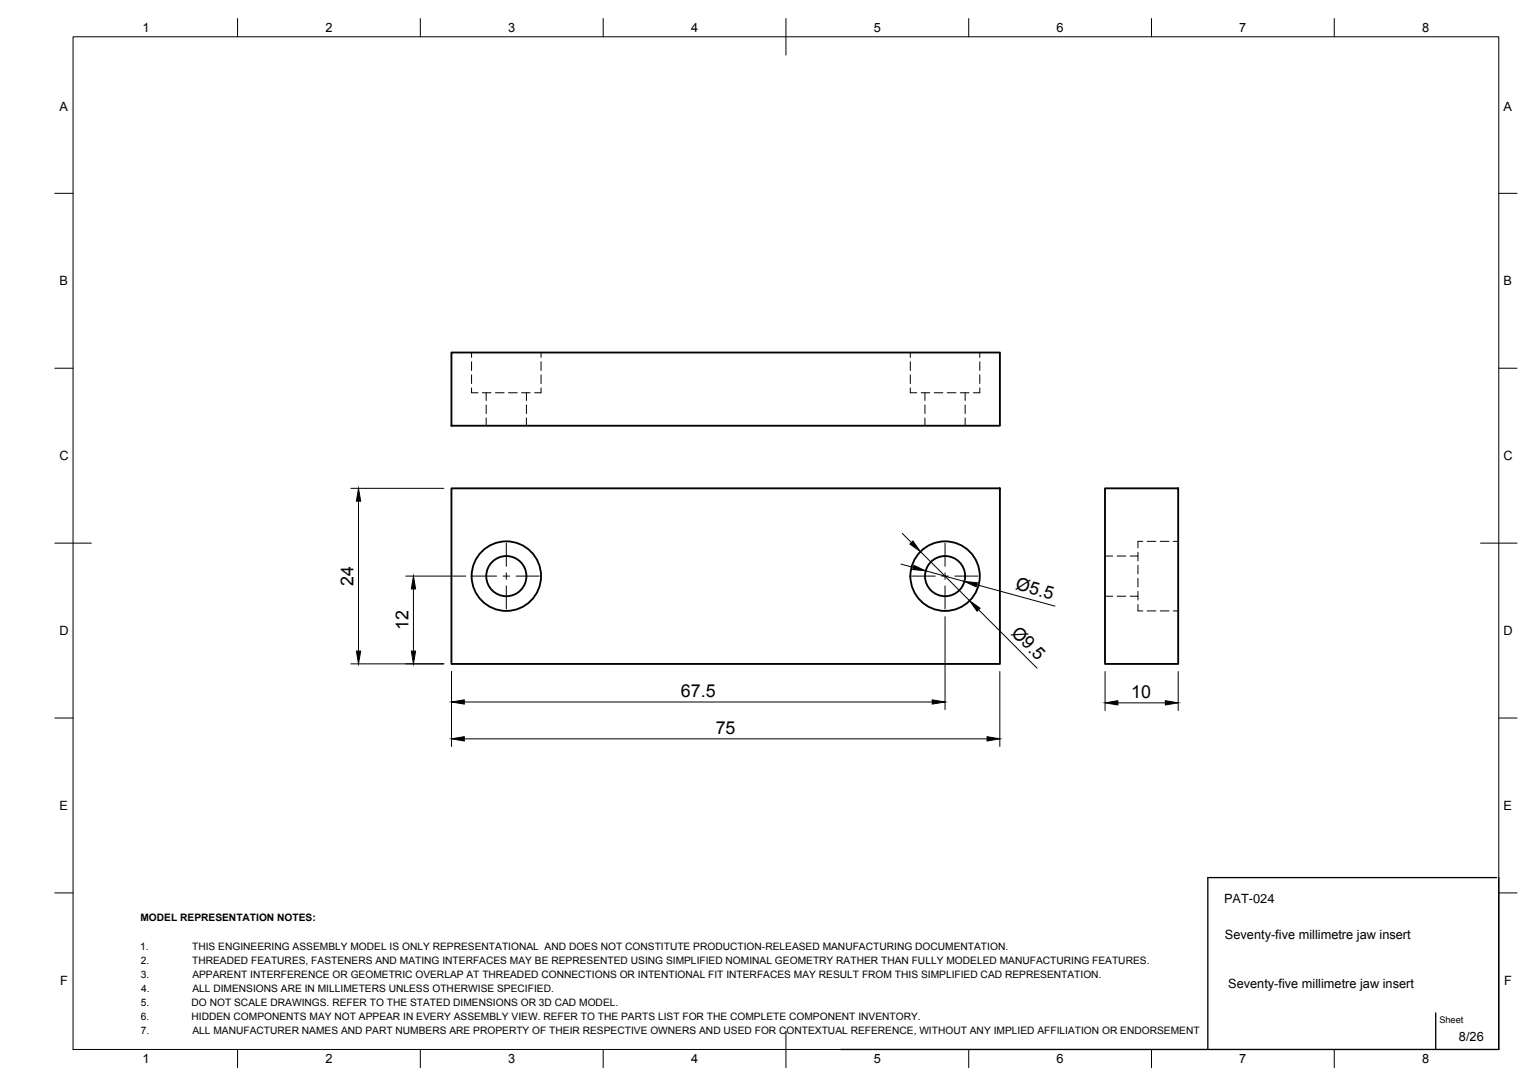
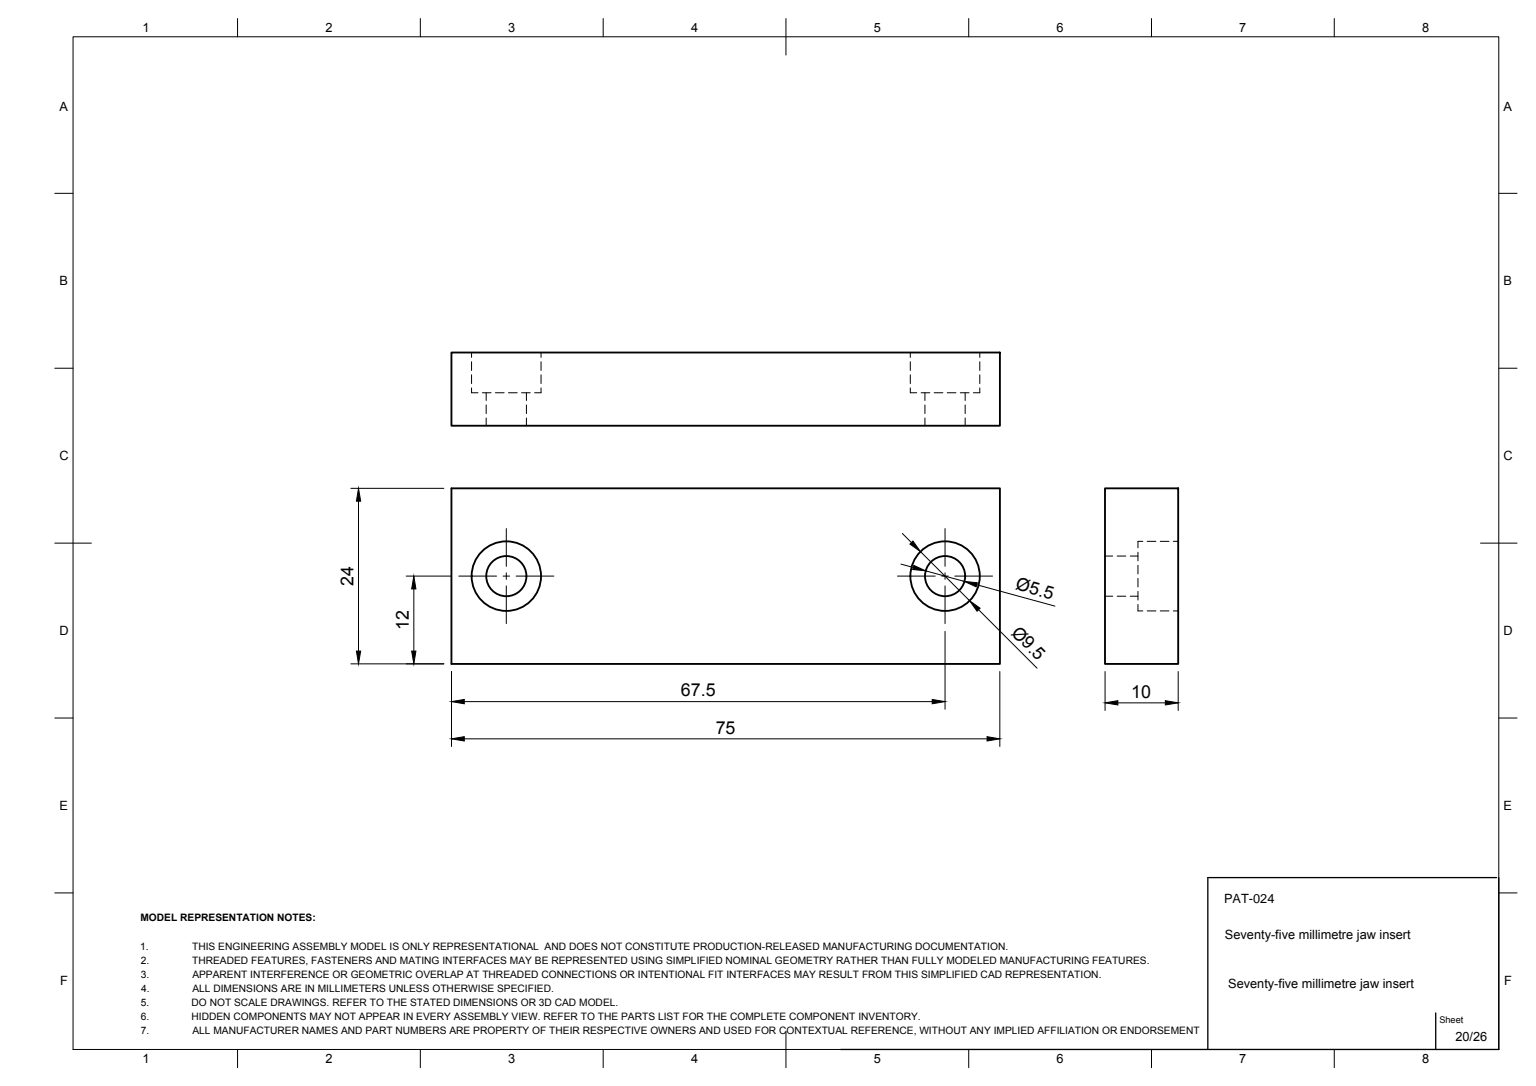
ISO-10303-21;
HEADER;
/* Generated by software containing ST-Developer
 * from STEP Tools, Inc. (www.steptools.com) 
 */

FILE_DESCRIPTION(
/* description */ ('Compact handwheel screw vise'),
/* implementation_level */ '2;1');

FILE_NAME(
/* name */ 'Seventy-five millimetre jaw insert.step',
/* time_stamp */ '2026-10-29T16:08:22-07:00',
/* author */ (''),
/* organization */ (''),
/* preprocessor_version */ 'ST-DEVELOPER v20.2',
/* originating_system */ 'Autodesk Translation Framework v15.17.0.0',
/* authorisation */ '');

FILE_SCHEMA (('AUTOMOTIVE_DESIGN { 1 0 10303 214 3 1 1 }'));
ENDSEC;

DATA;
#10=MECHANICAL_DESIGN_GEOMETRIC_PRESENTATION_REPRESENTATION('',(#649),#25074);
#593=SHAPE_REPRESENTATION_RELATIONSHIP('SRR','None',#25201,#621);
#621=ADVANCED_BREP_SHAPE_REPRESENTATION('',(#685),#25048);
#649=STYLED_ITEM('',(#25453),#685);
#685=MANIFOLD_SOLID_BREP('Body1',#8057);
#753=FACE_BOUND('',#1590,.T.);
#754=FACE_BOUND('',#1591,.T.);
#755=FACE_BOUND('',#1595,.T.);
#756=FACE_BOUND('',#1596,.T.);
#757=FACE_BOUND('',#1599,.T.);
#758=FACE_BOUND('',#1602,.T.);
#860=PLANE('',#8528);
#861=PLANE('',#8529);
#862=PLANE('',#8532);
#863=PLANE('',#8533);
#864=PLANE('',#8534);
#865=PLANE('',#8539);
#866=PLANE('',#8543);
#867=PLANE('',#8547);
#1077=FACE_OUTER_BOUND('',#1588,.T.);
#1078=FACE_OUTER_BOUND('',#1589,.T.);
#1079=FACE_OUTER_BOUND('',#1592,.T.);
#1080=FACE_OUTER_BOUND('',#1593,.T.);
#1081=FACE_OUTER_BOUND('',#1594,.T.);
#1082=FACE_OUTER_BOUND('',#1597,.T.);
#1083=FACE_OUTER_BOUND('',#1598,.T.);
#1084=FACE_OUTER_BOUND('',#1600,.T.);
#1085=FACE_OUTER_BOUND('',#1601,.T.);
#1086=FACE_OUTER_BOUND('',#1603,.T.);
#1087=FACE_OUTER_BOUND('',#1604,.T.);
#1088=FACE_OUTER_BOUND('',#1605,.T.);
#1588=EDGE_LOOP('',(#5423,#5424,#5425,#5426));
#1589=EDGE_LOOP('',(#5427,#5428,#5429,#5430));
#1590=EDGE_LOOP('',(#5431));
#1591=EDGE_LOOP('',(#5432));
#1592=EDGE_LOOP('',(#5433,#5434,#5435,#5436));
#1593=EDGE_LOOP('',(#5437,#5438,#5439,#5440));
#1594=EDGE_LOOP('',(#5441,#5442,#5443,#5444));
#1595=EDGE_LOOP('',(#5445));
#1596=EDGE_LOOP('',(#5446));
#1597=EDGE_LOOP('',(#5447,#5448,#5449,#5450));
#1598=EDGE_LOOP('',(#5451));
#1599=EDGE_LOOP('',(#5452));
#1600=EDGE_LOOP('',(#5453,#5454,#5455,#5456));
#1601=EDGE_LOOP('',(#5457));
#1602=EDGE_LOOP('',(#5458));
#1603=EDGE_LOOP('',(#5459,#5460,#5461,#5462));
#1604=EDGE_LOOP('',(#5463,#5464,#5465,#5466));
#1605=EDGE_LOOP('',(#5467,#5468,#5469,#5470));
#2140=LINE('',#11614,#2648);
#2141=LINE('',#11616,#2649);
#2142=LINE('',#11618,#2650);
#2143=LINE('',#11619,#2651);
#2144=LINE('',#11622,#2652);
#2145=LINE('',#11624,#2653);
#2146=LINE('',#11625,#2654);
#2147=LINE('',#11632,#2655);
#2148=LINE('',#11633,#2656);
#2149=LINE('',#11636,#2657);
#2150=LINE('',#11637,#2658);
#2151=LINE('',#11639,#2659);
#2152=LINE('',#11647,#2660);
#2153=LINE('',#11654,#2661);
#2154=LINE('',#11659,#2662);
#2155=LINE('',#11661,#2663);
#2648=VECTOR('',#9538,1.);
#2649=VECTOR('',#9539,1.);
#2650=VECTOR('',#9540,1.);
#2651=VECTOR('',#9541,1.);
#2652=VECTOR('',#9544,1.);
#2653=VECTOR('',#9545,1.);
#2654=VECTOR('',#9546,1.);
#2655=VECTOR('',#9553,1.);
#2656=VECTOR('',#9554,1.);
#2657=VECTOR('',#9557,1.);
#2658=VECTOR('',#9558,1.);
#2659=VECTOR('',#9561,1.);
#2660=VECTOR('',#9570,0.475);
#2661=VECTOR('',#9579,0.475);
#2662=VECTOR('',#9586,0.275);
#2663=VECTOR('',#9589,0.275);
#3132=CIRCLE('',#8530,0.275);
#3133=CIRCLE('',#8531,0.275);
#3134=CIRCLE('',#8535,0.475);
#3135=CIRCLE('',#8536,0.475);
#3136=CIRCLE('',#8538,0.475);
#3137=CIRCLE('',#8540,0.275);
#3138=CIRCLE('',#8542,0.475);
#3139=CIRCLE('',#8544,0.275);
#3421=VERTEX_POINT('',#11612);
#3422=VERTEX_POINT('',#11613);
#3423=VERTEX_POINT('',#11615);
#3424=VERTEX_POINT('',#11617);
#3425=VERTEX_POINT('',#11621);
#3426=VERTEX_POINT('',#11623);
#3427=VERTEX_POINT('',#11626);
#3428=VERTEX_POINT('',#11628);
#3429=VERTEX_POINT('',#11631);
#3430=VERTEX_POINT('',#11635);
#3431=VERTEX_POINT('',#11640);
#3432=VERTEX_POINT('',#11642);
#3433=VERTEX_POINT('',#11645);
#3434=VERTEX_POINT('',#11649);
#3435=VERTEX_POINT('',#11652);
#3436=VERTEX_POINT('',#11656);
#4198=EDGE_CURVE('',#3421,#3422,#2140,.T.);
#4199=EDGE_CURVE('',#3423,#3421,#2141,.T.);
#4200=EDGE_CURVE('',#3424,#3423,#2142,.T.);
#4201=EDGE_CURVE('',#3422,#3424,#2143,.T.);
#4202=EDGE_CURVE('',#3423,#3425,#2144,.T.);
#4203=EDGE_CURVE('',#3425,#3426,#2145,.T.);
#4204=EDGE_CURVE('',#3424,#3426,#2146,.T.);
#4205=EDGE_CURVE('',#3427,#3427,#3132,.T.);
#4206=EDGE_CURVE('',#3428,#3428,#3133,.T.);
#4207=EDGE_CURVE('',#3429,#3421,#2147,.T.);
#4208=EDGE_CURVE('',#3429,#3425,#2148,.T.);
#4209=EDGE_CURVE('',#3430,#3429,#2149,.T.);
#4210=EDGE_CURVE('',#3426,#3430,#2150,.T.);
#4211=EDGE_CURVE('',#3430,#3422,#2151,.T.);
#4212=EDGE_CURVE('',#3431,#3431,#3134,.T.);
#4213=EDGE_CURVE('',#3432,#3432,#3135,.T.);
#4214=EDGE_CURVE('',#3433,#3433,#3136,.T.);
#4215=EDGE_CURVE('',#3433,#3432,#2152,.T.);
#4216=EDGE_CURVE('',#3434,#3434,#3137,.T.);
#4217=EDGE_CURVE('',#3435,#3435,#3138,.T.);
#4218=EDGE_CURVE('',#3435,#3431,#2153,.T.);
#4219=EDGE_CURVE('',#3436,#3436,#3139,.T.);
#4220=EDGE_CURVE('',#3428,#3434,#2154,.T.);
#4221=EDGE_CURVE('',#3427,#3436,#2155,.T.);
#5423=ORIENTED_EDGE('',*,*,#4198,.F.);
#5424=ORIENTED_EDGE('',*,*,#4199,.F.);
#5425=ORIENTED_EDGE('',*,*,#4200,.F.);
#5426=ORIENTED_EDGE('',*,*,#4201,.F.);
#5427=ORIENTED_EDGE('',*,*,#4200,.T.);
#5428=ORIENTED_EDGE('',*,*,#4202,.T.);
#5429=ORIENTED_EDGE('',*,*,#4203,.T.);
#5430=ORIENTED_EDGE('',*,*,#4204,.F.);
#5431=ORIENTED_EDGE('',*,*,#4205,.T.);
#5432=ORIENTED_EDGE('',*,*,#4206,.T.);
#5433=ORIENTED_EDGE('',*,*,#4199,.T.);
#5434=ORIENTED_EDGE('',*,*,#4207,.F.);
#5435=ORIENTED_EDGE('',*,*,#4208,.T.);
#5436=ORIENTED_EDGE('',*,*,#4202,.F.);
#5437=ORIENTED_EDGE('',*,*,#4203,.F.);
#5438=ORIENTED_EDGE('',*,*,#4208,.F.);
#5439=ORIENTED_EDGE('',*,*,#4209,.F.);
#5440=ORIENTED_EDGE('',*,*,#4210,.F.);
#5441=ORIENTED_EDGE('',*,*,#4198,.T.);
#5442=ORIENTED_EDGE('',*,*,#4211,.F.);
#5443=ORIENTED_EDGE('',*,*,#4209,.T.);
#5444=ORIENTED_EDGE('',*,*,#4207,.T.);
#5445=ORIENTED_EDGE('',*,*,#4212,.T.);
#5446=ORIENTED_EDGE('',*,*,#4213,.T.);
#5447=ORIENTED_EDGE('',*,*,#4214,.F.);
#5448=ORIENTED_EDGE('',*,*,#4215,.T.);
#5449=ORIENTED_EDGE('',*,*,#4213,.F.);
#5450=ORIENTED_EDGE('',*,*,#4215,.F.);
#5451=ORIENTED_EDGE('',*,*,#4214,.T.);
#5452=ORIENTED_EDGE('',*,*,#4216,.F.);
#5453=ORIENTED_EDGE('',*,*,#4217,.F.);
#5454=ORIENTED_EDGE('',*,*,#4218,.T.);
#5455=ORIENTED_EDGE('',*,*,#4212,.F.);
#5456=ORIENTED_EDGE('',*,*,#4218,.F.);
#5457=ORIENTED_EDGE('',*,*,#4217,.T.);
#5458=ORIENTED_EDGE('',*,*,#4219,.F.);
#5459=ORIENTED_EDGE('',*,*,#4206,.F.);
#5460=ORIENTED_EDGE('',*,*,#4220,.T.);
#5461=ORIENTED_EDGE('',*,*,#4216,.T.);
#5462=ORIENTED_EDGE('',*,*,#4220,.F.);
#5463=ORIENTED_EDGE('',*,*,#4205,.F.);
#5464=ORIENTED_EDGE('',*,*,#4221,.T.);
#5465=ORIENTED_EDGE('',*,*,#4219,.T.);
#5466=ORIENTED_EDGE('',*,*,#4221,.F.);
#5467=ORIENTED_EDGE('',*,*,#4201,.T.);
#5468=ORIENTED_EDGE('',*,*,#4204,.T.);
#5469=ORIENTED_EDGE('',*,*,#4210,.T.);
#5470=ORIENTED_EDGE('',*,*,#4211,.T.);
#7372=CYLINDRICAL_SURFACE('',#8537,0.475);
#7373=CYLINDRICAL_SURFACE('',#8541,0.475);
#7374=CYLINDRICAL_SURFACE('',#8545,0.275);
#7375=CYLINDRICAL_SURFACE('',#8546,0.275);
#7647=ADVANCED_FACE('',(#1077),#860,.T.);
#7648=ADVANCED_FACE('',(#1078,#753,#754),#861,.T.);
#7649=ADVANCED_FACE('',(#1079),#862,.F.);
#7650=ADVANCED_FACE('',(#1080),#863,.F.);
#7651=ADVANCED_FACE('',(#1081,#755,#756),#864,.T.);
#7652=ADVANCED_FACE('',(#1082),#7372,.F.);
#7653=ADVANCED_FACE('',(#1083,#757),#865,.T.);
#7654=ADVANCED_FACE('',(#1084),#7373,.F.);
#7655=ADVANCED_FACE('',(#1085,#758),#866,.T.);
#7656=ADVANCED_FACE('',(#1086),#7374,.F.);
#7657=ADVANCED_FACE('',(#1087),#7375,.F.);
#7658=ADVANCED_FACE('',(#1088),#867,.T.);
#8057=CLOSED_SHELL('',(#7647,#7648,#7649,#7650,#7651,#7652,#7653,#7654,
#7655,#7656,#7657,#7658));
#8527=AXIS2_PLACEMENT_3D('',#11610,#9534,#9535);
#8528=AXIS2_PLACEMENT_3D('',#11611,#9536,#9537);
#8529=AXIS2_PLACEMENT_3D('',#11620,#9542,#9543);
#8530=AXIS2_PLACEMENT_3D('',#11627,#9547,#9548);
#8531=AXIS2_PLACEMENT_3D('',#11629,#9549,#9550);
#8532=AXIS2_PLACEMENT_3D('',#11630,#9551,#9552);
#8533=AXIS2_PLACEMENT_3D('',#11634,#9555,#9556);
#8534=AXIS2_PLACEMENT_3D('',#11638,#9559,#9560);
#8535=AXIS2_PLACEMENT_3D('',#11641,#9562,#9563);
#8536=AXIS2_PLACEMENT_3D('',#11643,#9564,#9565);
#8537=AXIS2_PLACEMENT_3D('',#11644,#9566,#9567);
#8538=AXIS2_PLACEMENT_3D('',#11646,#9568,#9569);
#8539=AXIS2_PLACEMENT_3D('',#11648,#9571,#9572);
#8540=AXIS2_PLACEMENT_3D('',#11650,#9573,#9574);
#8541=AXIS2_PLACEMENT_3D('',#11651,#9575,#9576);
#8542=AXIS2_PLACEMENT_3D('',#11653,#9577,#9578);
#8543=AXIS2_PLACEMENT_3D('',#11655,#9580,#9581);
#8544=AXIS2_PLACEMENT_3D('',#11657,#9582,#9583);
#8545=AXIS2_PLACEMENT_3D('',#11658,#9584,#9585);
#8546=AXIS2_PLACEMENT_3D('',#11660,#9587,#9588);
#8547=AXIS2_PLACEMENT_3D('',#11662,#9590,#9591);
#9534=DIRECTION('axis',(0.,0.,1.));
#9535=DIRECTION('refdir',(1.,0.,0.));
#9536=DIRECTION('center_axis',(0.,1.,0.));
#9537=DIRECTION('ref_axis',(1.,0.,0.));
#9538=DIRECTION('',(0.,0.,1.));
#9539=DIRECTION('',(1.,0.,0.));
#9540=DIRECTION('',(0.,0.,-1.));
#9541=DIRECTION('',(-1.,0.,0.));
#9542=DIRECTION('center_axis',(-1.,0.,0.));
#9543=DIRECTION('ref_axis',(0.,-1.,0.));
#9544=DIRECTION('',(0.,-1.,0.));
#9545=DIRECTION('',(0.,0.,1.));
#9546=DIRECTION('',(0.,-1.,0.));
#9547=DIRECTION('center_axis',(1.,0.,0.));
#9548=DIRECTION('ref_axis',(0.,0.,-1.));
#9549=DIRECTION('center_axis',(1.,0.,0.));
#9550=DIRECTION('ref_axis',(0.,0.,-1.));
#9551=DIRECTION('center_axis',(0.,0.,1.));
#9552=DIRECTION('ref_axis',(1.,0.,0.));
#9553=DIRECTION('',(0.,1.,0.));
#9554=DIRECTION('',(-1.,0.,0.));
#9555=DIRECTION('center_axis',(0.,1.,0.));
#9556=DIRECTION('ref_axis',(0.,0.,1.));
#9557=DIRECTION('',(0.,0.,-1.));
#9558=DIRECTION('',(1.,0.,0.));
#9559=DIRECTION('center_axis',(1.,0.,0.));
#9560=DIRECTION('ref_axis',(0.,1.,0.));
#9561=DIRECTION('',(0.,1.,0.));
#9562=DIRECTION('center_axis',(-1.,0.,0.));
#9563=DIRECTION('ref_axis',(0.,0.,-1.));
#9564=DIRECTION('center_axis',(-1.,0.,0.));
#9565=DIRECTION('ref_axis',(0.,0.,-1.));
#9566=DIRECTION('center_axis',(1.,0.,0.));
#9567=DIRECTION('ref_axis',(0.,0.,-1.));
#9568=DIRECTION('center_axis',(1.,0.,0.));
#9569=DIRECTION('ref_axis',(0.,0.,-1.));
#9570=DIRECTION('',(1.,0.,0.));
#9571=DIRECTION('center_axis',(1.,0.,0.));
#9572=DIRECTION('ref_axis',(0.,0.,-1.));
#9573=DIRECTION('center_axis',(1.,0.,0.));
#9574=DIRECTION('ref_axis',(0.,0.,-1.));
#9575=DIRECTION('center_axis',(1.,0.,0.));
#9576=DIRECTION('ref_axis',(0.,0.,-1.));
#9577=DIRECTION('center_axis',(1.,0.,0.));
#9578=DIRECTION('ref_axis',(0.,0.,-1.));
#9579=DIRECTION('',(1.,0.,0.));
#9580=DIRECTION('center_axis',(1.,0.,0.));
#9581=DIRECTION('ref_axis',(0.,0.,-1.));
#9582=DIRECTION('center_axis',(1.,0.,0.));
#9583=DIRECTION('ref_axis',(0.,0.,-1.));
#9584=DIRECTION('center_axis',(1.,0.,0.));
#9585=DIRECTION('ref_axis',(0.,0.,-1.));
#9586=DIRECTION('',(1.,0.,0.));
#9587=DIRECTION('center_axis',(1.,0.,0.));
#9588=DIRECTION('ref_axis',(0.,0.,-1.));
#9589=DIRECTION('',(1.,0.,0.));
#9590=DIRECTION('center_axis',(0.,0.,1.));
#9591=DIRECTION('ref_axis',(1.,0.,0.));
#11610=CARTESIAN_POINT('',(0.,0.,0.));
#11611=CARTESIAN_POINT('Origin',(14.95,3.75,5.));
#11612=CARTESIAN_POINT('',(4.,3.75,4.6));
#11613=CARTESIAN_POINT('',(4.,3.75,7.));
#11614=CARTESIAN_POINT('',(4.,3.75,4.8));
#11615=CARTESIAN_POINT('',(3.,3.75,4.6));
#11616=CARTESIAN_POINT('',(9.225,3.75,4.6));
#11617=CARTESIAN_POINT('',(3.,3.75,7.));
#11618=CARTESIAN_POINT('',(3.,3.75,4.8));
#11619=CARTESIAN_POINT('',(9.225,3.75,7.));
#11620=CARTESIAN_POINT('Origin',(3.,5.,4.6));
#11621=CARTESIAN_POINT('',(3.,-3.75,4.6));
#11622=CARTESIAN_POINT('',(3.,5.,4.6));
#11623=CARTESIAN_POINT('',(3.,-3.75,7.));
#11624=CARTESIAN_POINT('',(3.,-3.75,4.8));
#11625=CARTESIAN_POINT('',(3.,5.,7.));
#11626=CARTESIAN_POINT('',(3.,3.,6.075));
#11627=CARTESIAN_POINT('Origin',(3.,3.,5.8));
#11628=CARTESIAN_POINT('',(3.,-3.,6.075));
#11629=CARTESIAN_POINT('Origin',(3.,-3.,5.8));
#11630=CARTESIAN_POINT('Origin',(3.5,0.,4.6));
#11631=CARTESIAN_POINT('',(4.,-3.75,4.6));
#11632=CARTESIAN_POINT('',(4.,-5.,4.6));
#11633=CARTESIAN_POINT('',(9.225,-3.75,4.6));
#11634=CARTESIAN_POINT('Origin',(14.95,-3.75,5.));
#11635=CARTESIAN_POINT('',(4.,-3.75,7.));
#11636=CARTESIAN_POINT('',(4.,-3.75,4.8));
#11637=CARTESIAN_POINT('',(9.225,-3.75,7.));
#11638=CARTESIAN_POINT('Origin',(4.,-5.,4.6));
#11639=CARTESIAN_POINT('',(4.,-5.,7.));
#11640=CARTESIAN_POINT('',(4.,3.,6.275));
#11641=CARTESIAN_POINT('Origin',(4.,3.,5.8));
#11642=CARTESIAN_POINT('',(4.,-3.,6.275));
#11643=CARTESIAN_POINT('Origin',(4.,-3.,5.8));
#11644=CARTESIAN_POINT('Origin',(3.45,-3.,5.8));
#11645=CARTESIAN_POINT('',(3.45,-3.,6.275));
#11646=CARTESIAN_POINT('Origin',(3.45,-3.,5.8));
#11647=CARTESIAN_POINT('',(3.45,-3.,6.275));
#11648=CARTESIAN_POINT('Origin',(3.45,-3.,5.8));
#11649=CARTESIAN_POINT('',(3.45,-3.,6.075));
#11650=CARTESIAN_POINT('Origin',(3.45,-3.,5.8));
#11651=CARTESIAN_POINT('Origin',(3.45,3.,5.8));
#11652=CARTESIAN_POINT('',(3.45,3.,6.275));
#11653=CARTESIAN_POINT('Origin',(3.45,3.,5.8));
#11654=CARTESIAN_POINT('',(3.45,3.,6.275));
#11655=CARTESIAN_POINT('Origin',(3.45,3.,5.8));
#11656=CARTESIAN_POINT('',(3.45,3.,6.075));
#11657=CARTESIAN_POINT('Origin',(3.45,3.,5.8));
#11658=CARTESIAN_POINT('Origin',(2.9,-3.,5.8));
#11659=CARTESIAN_POINT('',(2.9,-3.,6.075));
#11660=CARTESIAN_POINT('Origin',(2.9,3.,5.8));
#11661=CARTESIAN_POINT('',(2.9,3.,6.075));
#11662=CARTESIAN_POINT('Origin',(3.5,0.,7.));
#25014=UNCERTAINTY_MEASURE_WITH_UNIT(LENGTH_MEASURE(0.001),#25075,
'DISTANCE_ACCURACY_VALUE',
'Maximum model space distance between geometric entities at asserted c
onnectivities');
#25040=UNCERTAINTY_MEASURE_WITH_UNIT(LENGTH_MEASURE(0.001),#25075,
'DISTANCE_ACCURACY_VALUE',
'Maximum model space distance between geometric entities at asserted c
onnectivities');
#25048=(
GEOMETRIC_REPRESENTATION_CONTEXT(3)
GLOBAL_UNCERTAINTY_ASSIGNED_CONTEXT((#25014))
GLOBAL_UNIT_ASSIGNED_CONTEXT((#25075,#25077,#25078))
REPRESENTATION_CONTEXT('','3D')
);
#25074=(
GEOMETRIC_REPRESENTATION_CONTEXT(3)
GLOBAL_UNCERTAINTY_ASSIGNED_CONTEXT((#25040))
GLOBAL_UNIT_ASSIGNED_CONTEXT((#25075,#25077,#25078))
REPRESENTATION_CONTEXT('','3D')
);
#25075=(
LENGTH_UNIT()
NAMED_UNIT(*)
SI_UNIT(.CENTI.,.METRE.)
);
#25077=(
NAMED_UNIT(*)
PLANE_ANGLE_UNIT()
SI_UNIT($,.RADIAN.)
);
#25078=(
NAMED_UNIT(*)
SI_UNIT($,.STERADIAN.)
SOLID_ANGLE_UNIT()
);
#25086=SHAPE_DEFINITION_REPRESENTATION(#25119,#25201);
#25119=PRODUCT_DEFINITION_SHAPE('',$,#25235);
#25201=SHAPE_REPRESENTATION('',(#8527),#25048);
#25227=PRODUCT_DEFINITION_CONTEXT('part definition',#25328,'design');
#25235=PRODUCT_DEFINITION('Seventy-five millimetre jaw insert',
'Seventy-five millimetre jaw insert',#25268,#25227);
#25268=PRODUCT_DEFINITION_FORMATION('',$,#25337);
#25328=APPLICATION_CONTEXT(
'Core Data for Automotive Mechanical Design Process');
#25329=PRODUCT_CONTEXT('part definition',#25328,'mechanical');
#25337=PRODUCT('Seventy-five millimetre jaw insert',
'Seventy-five millimetre jaw insert',
'Seventy-five millimetre jaw insert',(#25329));
#25447=COLOUR_RGB('Off White',0.89,0.88,0.83);
#25448=FILL_AREA_STYLE_COLOUR('',#25447);
#25449=FILL_AREA_STYLE('',(#25448));
#25450=SURFACE_STYLE_FILL_AREA(#25449);
#25451=SURFACE_SIDE_STYLE('',(#25450));
#25452=SURFACE_STYLE_USAGE(.BOTH.,#25451);
#25453=PRESENTATION_STYLE_ASSIGNMENT((#25452));
ENDSEC;
END-ISO-10303-21;
